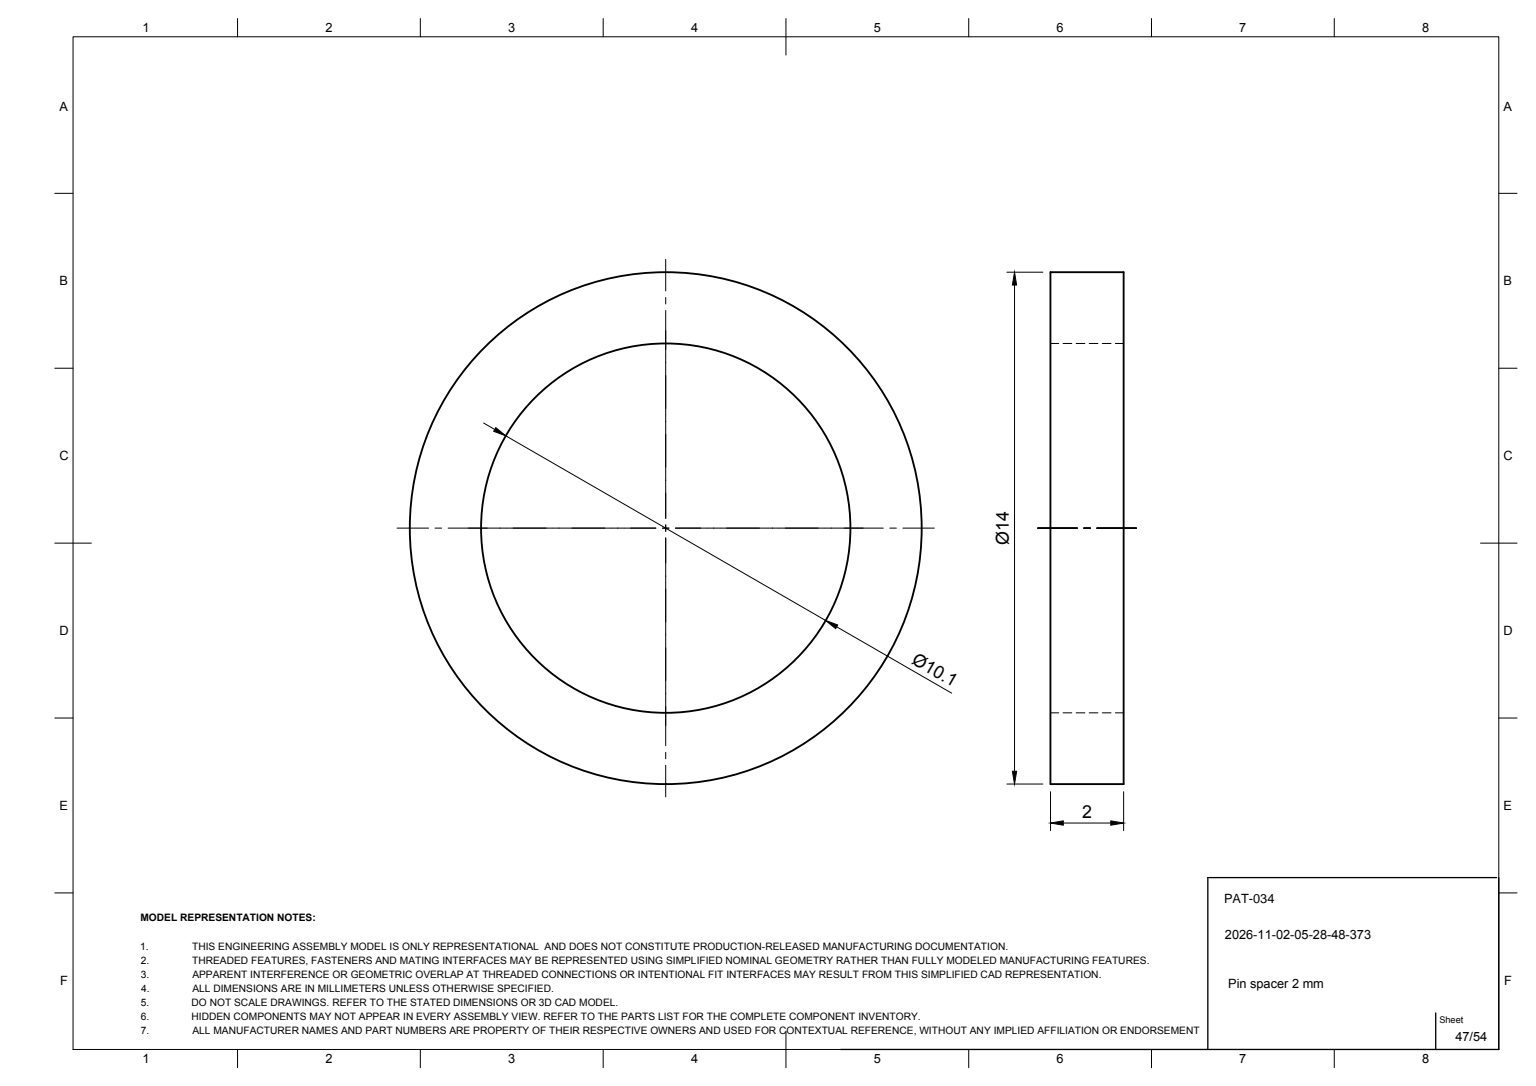
ISO-10303-21;
HEADER;
/* Generated by software containing ST-Developer
 * from STEP Tools, Inc. (www.steptools.com) 
 */

FILE_DESCRIPTION(
/* description */ ('Fatigue rig crank-slider'),
/* implementation_level */ '2;1');

FILE_NAME(
/* name */ 'Pin spacer 2 mm.step',
/* time_stamp */ '2026-10-28T03:24:50-07:00',
/* author */ (''),
/* organization */ (''),
/* preprocessor_version */ 'ST-DEVELOPER v20.2',
/* originating_system */ 'Autodesk Translation Framework v15.17.0.0',
/* authorisation */ '');

FILE_SCHEMA (('AUTOMOTIVE_DESIGN { 1 0 10303 214 3 1 1 }'));
ENDSEC;

DATA;
#10=MECHANICAL_DESIGN_GEOMETRIC_PRESENTATION_REPRESENTATION('',(#636),#16911);
#527=SHAPE_REPRESENTATION_RELATIONSHIP('SRR','None',#17171,#577);
#577=ADVANCED_BREP_SHAPE_REPRESENTATION('',(#693),#16900);
#636=STYLED_ITEM('',(#17487),#693);
#693=MANIFOLD_SOLID_BREP('Body1',#8929);
#882=FACE_BOUND('',#2340,.T.);
#883=FACE_BOUND('',#2342,.T.);
#1138=PLANE('',#10321);
#1139=PLANE('',#10322);
#1632=FACE_OUTER_BOUND('',#2337,.T.);
#1633=FACE_OUTER_BOUND('',#2338,.T.);
#1634=FACE_OUTER_BOUND('',#2339,.T.);
#1635=FACE_OUTER_BOUND('',#2341,.T.);
#2337=EDGE_LOOP('',(#7720,#7721,#7722,#7723));
#2338=EDGE_LOOP('',(#7724,#7725,#7726,#7727));
#2339=EDGE_LOOP('',(#7728));
#2340=EDGE_LOOP('',(#7729));
#2341=EDGE_LOOP('',(#7730));
#2342=EDGE_LOOP('',(#7731));
#2923=LINE('',#16209,#3569);
#2924=LINE('',#16215,#3570);
#3569=VECTOR('',#12677,0.505000000000001);
#3570=VECTOR('',#12684,0.699999999999999);
#4097=CIRCLE('',#10316,0.505000000000001);
#4098=CIRCLE('',#10317,0.505000000000001);
#4099=CIRCLE('',#10319,0.699999999999999);
#4100=CIRCLE('',#10320,0.699999999999999);
#4741=VERTEX_POINT('',#16206);
#4742=VERTEX_POINT('',#16208);
#4743=VERTEX_POINT('',#16212);
#4744=VERTEX_POINT('',#16214);
#5758=EDGE_CURVE('',#4741,#4741,#4097,.T.);
#5759=EDGE_CURVE('',#4741,#4742,#2923,.T.);
#5760=EDGE_CURVE('',#4742,#4742,#4098,.T.);
#5761=EDGE_CURVE('',#4743,#4743,#4099,.T.);
#5762=EDGE_CURVE('',#4743,#4744,#2924,.T.);
#5763=EDGE_CURVE('',#4744,#4744,#4100,.T.);
#7720=ORIENTED_EDGE('',*,*,#5758,.F.);
#7721=ORIENTED_EDGE('',*,*,#5759,.T.);
#7722=ORIENTED_EDGE('',*,*,#5760,.T.);
#7723=ORIENTED_EDGE('',*,*,#5759,.F.);
#7724=ORIENTED_EDGE('',*,*,#5761,.F.);
#7725=ORIENTED_EDGE('',*,*,#5762,.T.);
#7726=ORIENTED_EDGE('',*,*,#5763,.T.);
#7727=ORIENTED_EDGE('',*,*,#5762,.F.);
#7728=ORIENTED_EDGE('',*,*,#5761,.T.);
#7729=ORIENTED_EDGE('',*,*,#5758,.T.);
#7730=ORIENTED_EDGE('',*,*,#5763,.F.);
#7731=ORIENTED_EDGE('',*,*,#5760,.F.);
#8337=CYLINDRICAL_SURFACE('',#10315,0.505000000000001);
#8338=CYLINDRICAL_SURFACE('',#10318,0.699999999999999);
#8770=ADVANCED_FACE('',(#1632),#8337,.F.);
#8771=ADVANCED_FACE('',(#1633),#8338,.T.);
#8772=ADVANCED_FACE('',(#1634,#882),#1138,.T.);
#8773=ADVANCED_FACE('',(#1635,#883),#1139,.F.);
#8929=CLOSED_SHELL('',(#8770,#8771,#8772,#8773));
#10314=AXIS2_PLACEMENT_3D('',#16204,#12671,#12672);
#10315=AXIS2_PLACEMENT_3D('',#16205,#12673,#12674);
#10316=AXIS2_PLACEMENT_3D('',#16207,#12675,#12676);
#10317=AXIS2_PLACEMENT_3D('',#16210,#12678,#12679);
#10318=AXIS2_PLACEMENT_3D('',#16211,#12680,#12681);
#10319=AXIS2_PLACEMENT_3D('',#16213,#12682,#12683);
#10320=AXIS2_PLACEMENT_3D('',#16216,#12685,#12686);
#10321=AXIS2_PLACEMENT_3D('',#16217,#12687,#12688);
#10322=AXIS2_PLACEMENT_3D('',#16218,#12689,#12690);
#12671=DIRECTION('axis',(0.,0.,1.));
#12672=DIRECTION('refdir',(1.,0.,0.));
#12673=DIRECTION('center_axis',(0.,1.,0.));
#12674=DIRECTION('ref_axis',(1.,0.,0.));
#12675=DIRECTION('center_axis',(0.,-1.,0.));
#12676=DIRECTION('ref_axis',(1.,0.,0.));
#12677=DIRECTION('',(0.,-1.,0.));
#12678=DIRECTION('center_axis',(0.,-1.,0.));
#12679=DIRECTION('ref_axis',(1.,0.,0.));
#12680=DIRECTION('center_axis',(0.,1.,0.));
#12681=DIRECTION('ref_axis',(1.,0.,0.));
#12682=DIRECTION('center_axis',(0.,1.,0.));
#12683=DIRECTION('ref_axis',(1.,0.,0.));
#12684=DIRECTION('',(0.,-1.,0.));
#12685=DIRECTION('center_axis',(0.,1.,0.));
#12686=DIRECTION('ref_axis',(1.,0.,0.));
#12687=DIRECTION('center_axis',(0.,1.,0.));
#12688=DIRECTION('ref_axis',(1.,0.,0.));
#12689=DIRECTION('center_axis',(0.,1.,0.));
#12690=DIRECTION('ref_axis',(1.,0.,0.));
#16204=CARTESIAN_POINT('',(0.,0.,0.));
#16205=CARTESIAN_POINT('Origin',(11.,3.3,12.));
#16206=CARTESIAN_POINT('',(10.495,3.5,12.));
#16207=CARTESIAN_POINT('Origin',(11.,3.5,12.));
#16208=CARTESIAN_POINT('',(10.495,3.3,12.));
#16209=CARTESIAN_POINT('',(10.495,3.3,12.));
#16210=CARTESIAN_POINT('Origin',(11.,3.3,12.));
#16211=CARTESIAN_POINT('Origin',(11.,3.3,12.));
#16212=CARTESIAN_POINT('',(10.3,3.5,12.));
#16213=CARTESIAN_POINT('Origin',(11.,3.5,12.));
#16214=CARTESIAN_POINT('',(10.3,3.3,12.));
#16215=CARTESIAN_POINT('',(10.3,3.3,12.));
#16216=CARTESIAN_POINT('Origin',(11.,3.3,12.));
#16217=CARTESIAN_POINT('Origin',(11.,3.5,12.));
#16218=CARTESIAN_POINT('Origin',(11.,3.3,12.));
#16841=UNCERTAINTY_MEASURE_WITH_UNIT(LENGTH_MEASURE(0.001),#16912,
'DISTANCE_ACCURACY_VALUE',
'Maximum model space distance between geometric entities at asserted c
onnectivities');
#16852=UNCERTAINTY_MEASURE_WITH_UNIT(LENGTH_MEASURE(0.001),#16912,
'DISTANCE_ACCURACY_VALUE',
'Maximum model space distance between geometric entities at asserted c
onnectivities');
#16900=(
GEOMETRIC_REPRESENTATION_CONTEXT(3)
GLOBAL_UNCERTAINTY_ASSIGNED_CONTEXT((#16841))
GLOBAL_UNIT_ASSIGNED_CONTEXT((#16912,#16914,#16915))
REPRESENTATION_CONTEXT('','3D')
);
#16911=(
GEOMETRIC_REPRESENTATION_CONTEXT(3)
GLOBAL_UNCERTAINTY_ASSIGNED_CONTEXT((#16852))
GLOBAL_UNIT_ASSIGNED_CONTEXT((#16912,#16914,#16915))
REPRESENTATION_CONTEXT('','3D')
);
#16912=(
LENGTH_UNIT()
NAMED_UNIT(*)
SI_UNIT(.CENTI.,.METRE.)
);
#16914=(
NAMED_UNIT(*)
PLANE_ANGLE_UNIT()
SI_UNIT($,.RADIAN.)
);
#16915=(
NAMED_UNIT(*)
SI_UNIT($,.STERADIAN.)
SOLID_ANGLE_UNIT()
);
#16963=SHAPE_DEFINITION_REPRESENTATION(#17035,#17171);
#17035=PRODUCT_DEFINITION_SHAPE('',$,#17230);
#17171=SHAPE_REPRESENTATION('',(#10314),#16900);
#17182=PRODUCT_DEFINITION_CONTEXT('part definition',#17358,'design');
#17230=PRODUCT_DEFINITION('Pin spacer 2 mm','Pin spacer 2 mm',#17288,#17182);
#17288=PRODUCT_DEFINITION_FORMATION('',$,#17407);
#17358=APPLICATION_CONTEXT(
'Core Data for Automotive Mechanical Design Process');
#17359=PRODUCT_CONTEXT('part definition',#17358,'mechanical');
#17407=PRODUCT('Pin spacer 2 mm','Pin spacer 2 mm','Pin spacer 2 mm',(#17359));
#17481=COLOUR_RGB('Grey',0.48,0.52,0.57);
#17482=FILL_AREA_STYLE_COLOUR('',#17481);
#17483=FILL_AREA_STYLE('',(#17482));
#17484=SURFACE_STYLE_FILL_AREA(#17483);
#17485=SURFACE_SIDE_STYLE('',(#17484));
#17486=SURFACE_STYLE_USAGE(.BOTH.,#17485);
#17487=PRESENTATION_STYLE_ASSIGNMENT((#17486));
ENDSEC;
END-ISO-10303-21;
